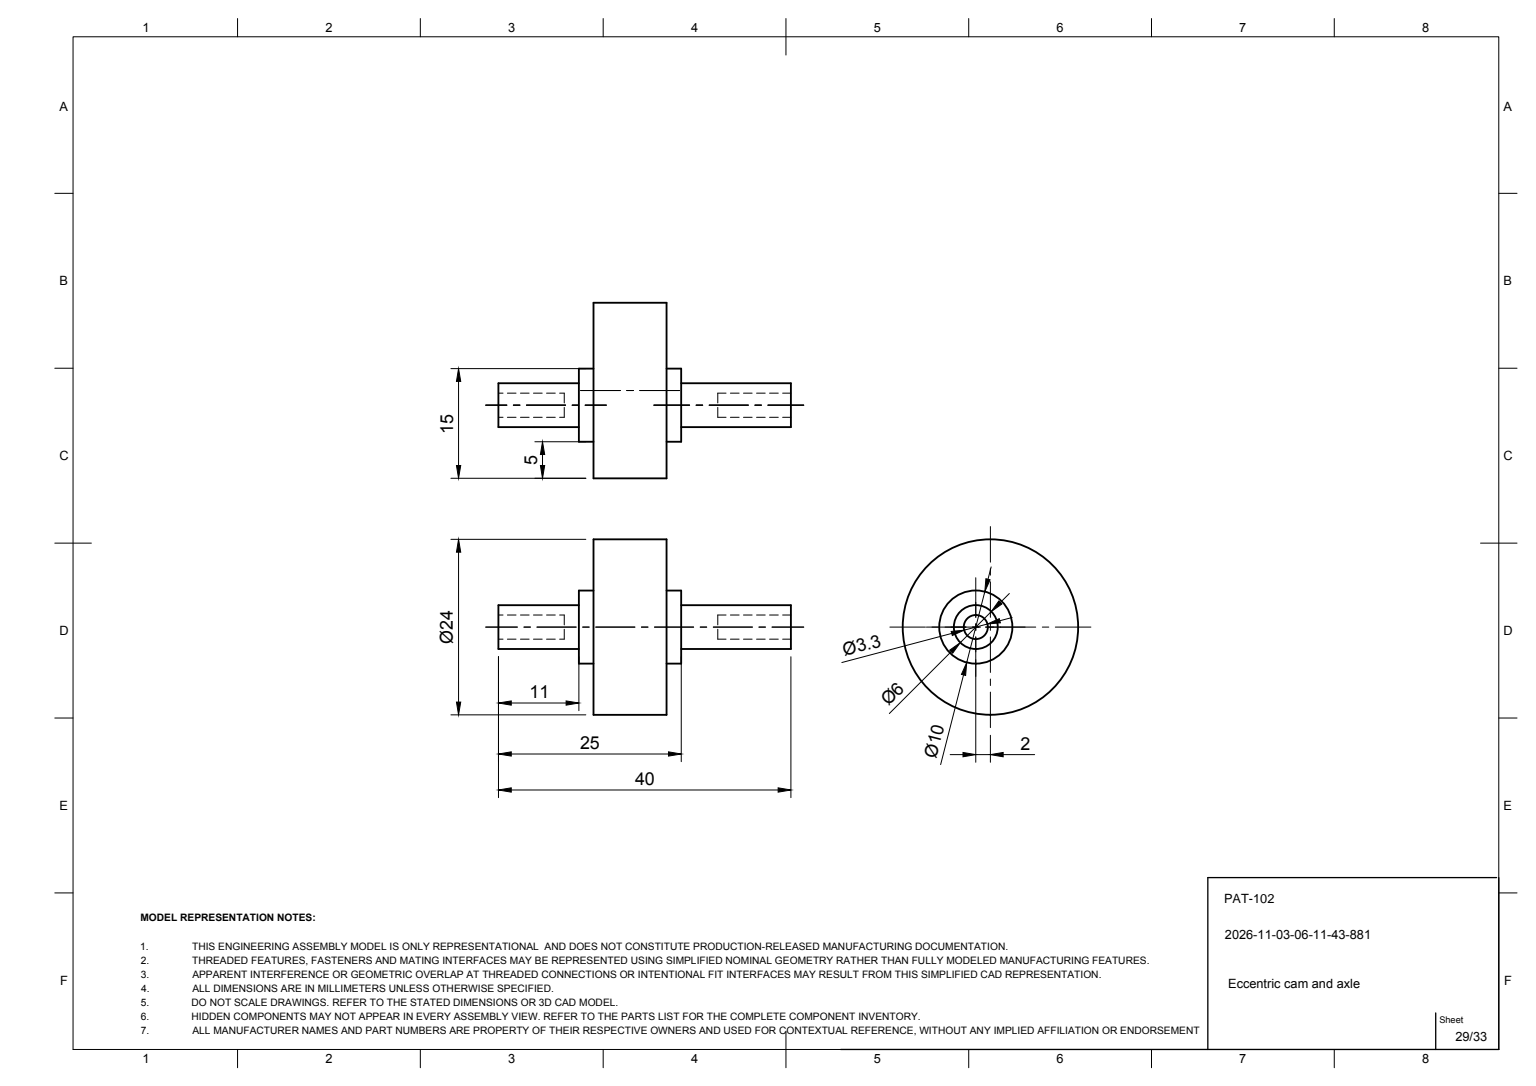
ISO-10303-21;
HEADER;
/* Generated by software containing ST-Developer
 * from STEP Tools, Inc. (www.steptools.com) 
 */

FILE_DESCRIPTION(
/* description */ ('Swing-away clamp arm'),
/* implementation_level */ '2;1');

FILE_NAME(
/* name */ 'Eccentric cam and axle.step',
/* time_stamp */ '2026-10-28T03:26:03-07:00',
/* author */ (''),
/* organization */ (''),
/* preprocessor_version */ 'ST-DEVELOPER v20.2',
/* originating_system */ 'Autodesk Translation Framework v15.17.0.0',
/* authorisation */ '');

FILE_SCHEMA (('AUTOMOTIVE_DESIGN { 1 0 10303 214 3 1 1 }'));
ENDSEC;

DATA;
#10=MECHANICAL_DESIGN_GEOMETRIC_PRESENTATION_REPRESENTATION('',(#320),#10627);
#260=SHAPE_REPRESENTATION_RELATIONSHIP('SRR','None',#10761,#286);
#286=ADVANCED_BREP_SHAPE_REPRESENTATION('',(#353),#10620);
#320=STYLED_ITEM('',(#10965),#353);
#353=MANIFOLD_SOLID_BREP('Body1',#4927);
#441=FACE_BOUND('',#1269,.T.);
#442=FACE_BOUND('',#1272,.T.);
#443=FACE_BOUND('',#1277,.T.);
#444=FACE_BOUND('',#1279,.T.);
#445=FACE_BOUND('',#1282,.T.);
#446=FACE_BOUND('',#1284,.T.);
#595=PLANE('',#5718);
#596=PLANE('',#5722);
#597=PLANE('',#5723);
#598=PLANE('',#5728);
#599=PLANE('',#5737);
#600=PLANE('',#5738);
#601=PLANE('',#5742);
#602=PLANE('',#5743);
#874=FACE_OUTER_BOUND('',#1264,.T.);
#875=FACE_OUTER_BOUND('',#1265,.T.);
#876=FACE_OUTER_BOUND('',#1266,.T.);
#877=FACE_OUTER_BOUND('',#1267,.T.);
#878=FACE_OUTER_BOUND('',#1268,.T.);
#879=FACE_OUTER_BOUND('',#1270,.T.);
#880=FACE_OUTER_BOUND('',#1271,.T.);
#881=FACE_OUTER_BOUND('',#1273,.T.);
#882=FACE_OUTER_BOUND('',#1274,.T.);
#883=FACE_OUTER_BOUND('',#1275,.T.);
#884=FACE_OUTER_BOUND('',#1276,.T.);
#885=FACE_OUTER_BOUND('',#1278,.T.);
#886=FACE_OUTER_BOUND('',#1280,.T.);
#887=FACE_OUTER_BOUND('',#1281,.T.);
#888=FACE_OUTER_BOUND('',#1283,.T.);
#1264=EDGE_LOOP('',(#4253,#4254,#4255,#4256));
#1265=EDGE_LOOP('',(#4257));
#1266=EDGE_LOOP('',(#4258,#4259,#4260,#4261));
#1267=EDGE_LOOP('',(#4262));
#1268=EDGE_LOOP('',(#4263));
#1269=EDGE_LOOP('',(#4264));
#1270=EDGE_LOOP('',(#4265,#4266,#4267,#4268));
#1271=EDGE_LOOP('',(#4269));
#1272=EDGE_LOOP('',(#4270));
#1273=EDGE_LOOP('',(#4271,#4272,#4273,#4274));
#1274=EDGE_LOOP('',(#4275,#4276,#4277,#4278));
#1275=EDGE_LOOP('',(#4279,#4280,#4281,#4282));
#1276=EDGE_LOOP('',(#4283));
#1277=EDGE_LOOP('',(#4284));
#1278=EDGE_LOOP('',(#4285));
#1279=EDGE_LOOP('',(#4286));
#1280=EDGE_LOOP('',(#4287,#4288,#4289,#4290));
#1281=EDGE_LOOP('',(#4291));
#1282=EDGE_LOOP('',(#4292));
#1283=EDGE_LOOP('',(#4293));
#1284=EDGE_LOOP('',(#4294));
#1602=LINE('',#10263,#1924);
#1603=LINE('',#10270,#1925);
#1604=LINE('',#10280,#1926);
#1605=LINE('',#10290,#1927);
#1606=LINE('',#10293,#1928);
#1607=LINE('',#10298,#1929);
#1608=LINE('',#10305,#1930);
#1924=VECTOR('',#7109,0.165);
#1925=VECTOR('',#7118,0.165);
#1926=VECTOR('',#7131,0.5);
#1927=VECTOR('',#7144,0.5);
#1928=VECTOR('',#7147,0.3);
#1929=VECTOR('',#7154,0.3);
#1930=VECTOR('',#7163,1.2);
#2211=CIRCLE('',#5716,0.165);
#2212=CIRCLE('',#5717,0.165);
#2213=CIRCLE('',#5720,0.165);
#2214=CIRCLE('',#5721,0.165);
#2215=CIRCLE('',#5724,0.5);
#2216=CIRCLE('',#5725,0.3);
#2217=CIRCLE('',#5727,0.5);
#2218=CIRCLE('',#5729,0.5);
#2219=CIRCLE('',#5730,0.3);
#2220=CIRCLE('',#5732,0.5);
#2221=CIRCLE('',#5734,0.3);
#2222=CIRCLE('',#5736,0.3);
#2223=CIRCLE('',#5740,1.2);
#2224=CIRCLE('',#5741,1.2);
#2594=VERTEX_POINT('',#10260);
#2595=VERTEX_POINT('',#10262);
#2596=VERTEX_POINT('',#10267);
#2597=VERTEX_POINT('',#10269);
#2598=VERTEX_POINT('',#10274);
#2599=VERTEX_POINT('',#10276);
#2600=VERTEX_POINT('',#10279);
#2601=VERTEX_POINT('',#10283);
#2602=VERTEX_POINT('',#10285);
#2603=VERTEX_POINT('',#10288);
#2604=VERTEX_POINT('',#10292);
#2605=VERTEX_POINT('',#10296);
#2606=VERTEX_POINT('',#10302);
#2607=VERTEX_POINT('',#10304);
#3159=EDGE_CURVE('',#2594,#2594,#2211,.T.);
#3160=EDGE_CURVE('',#2594,#2595,#1602,.T.);
#3161=EDGE_CURVE('',#2595,#2595,#2212,.T.);
#3162=EDGE_CURVE('',#2596,#2596,#2213,.T.);
#3163=EDGE_CURVE('',#2596,#2597,#1603,.T.);
#3164=EDGE_CURVE('',#2597,#2597,#2214,.T.);
#3165=EDGE_CURVE('',#2598,#2598,#2215,.T.);
#3166=EDGE_CURVE('',#2599,#2599,#2216,.T.);
#3167=EDGE_CURVE('',#2598,#2600,#1604,.T.);
#3168=EDGE_CURVE('',#2600,#2600,#2217,.T.);
#3169=EDGE_CURVE('',#2601,#2601,#2218,.T.);
#3170=EDGE_CURVE('',#2602,#2602,#2219,.T.);
#3171=EDGE_CURVE('',#2603,#2603,#2220,.T.);
#3172=EDGE_CURVE('',#2603,#2601,#1605,.T.);
#3173=EDGE_CURVE('',#2602,#2604,#1606,.T.);
#3174=EDGE_CURVE('',#2604,#2604,#2221,.T.);
#3175=EDGE_CURVE('',#2605,#2605,#2222,.T.);
#3176=EDGE_CURVE('',#2605,#2599,#1607,.T.);
#3177=EDGE_CURVE('',#2606,#2606,#2223,.T.);
#3178=EDGE_CURVE('',#2606,#2607,#1608,.T.);
#3179=EDGE_CURVE('',#2607,#2607,#2224,.T.);
#4253=ORIENTED_EDGE('',*,*,#3159,.F.);
#4254=ORIENTED_EDGE('',*,*,#3160,.T.);
#4255=ORIENTED_EDGE('',*,*,#3161,.F.);
#4256=ORIENTED_EDGE('',*,*,#3160,.F.);
#4257=ORIENTED_EDGE('',*,*,#3159,.T.);
#4258=ORIENTED_EDGE('',*,*,#3162,.F.);
#4259=ORIENTED_EDGE('',*,*,#3163,.T.);
#4260=ORIENTED_EDGE('',*,*,#3164,.T.);
#4261=ORIENTED_EDGE('',*,*,#3163,.F.);
#4262=ORIENTED_EDGE('',*,*,#3164,.F.);
#4263=ORIENTED_EDGE('',*,*,#3165,.T.);
#4264=ORIENTED_EDGE('',*,*,#3166,.F.);
#4265=ORIENTED_EDGE('',*,*,#3165,.F.);
#4266=ORIENTED_EDGE('',*,*,#3167,.T.);
#4267=ORIENTED_EDGE('',*,*,#3168,.F.);
#4268=ORIENTED_EDGE('',*,*,#3167,.F.);
#4269=ORIENTED_EDGE('',*,*,#3169,.F.);
#4270=ORIENTED_EDGE('',*,*,#3170,.F.);
#4271=ORIENTED_EDGE('',*,*,#3171,.F.);
#4272=ORIENTED_EDGE('',*,*,#3172,.T.);
#4273=ORIENTED_EDGE('',*,*,#3169,.T.);
#4274=ORIENTED_EDGE('',*,*,#3172,.F.);
#4275=ORIENTED_EDGE('',*,*,#3170,.T.);
#4276=ORIENTED_EDGE('',*,*,#3173,.T.);
#4277=ORIENTED_EDGE('',*,*,#3174,.T.);
#4278=ORIENTED_EDGE('',*,*,#3173,.F.);
#4279=ORIENTED_EDGE('',*,*,#3175,.F.);
#4280=ORIENTED_EDGE('',*,*,#3176,.T.);
#4281=ORIENTED_EDGE('',*,*,#3166,.T.);
#4282=ORIENTED_EDGE('',*,*,#3176,.F.);
#4283=ORIENTED_EDGE('',*,*,#3175,.T.);
#4284=ORIENTED_EDGE('',*,*,#3161,.T.);
#4285=ORIENTED_EDGE('',*,*,#3174,.F.);
#4286=ORIENTED_EDGE('',*,*,#3162,.T.);
#4287=ORIENTED_EDGE('',*,*,#3177,.F.);
#4288=ORIENTED_EDGE('',*,*,#3178,.T.);
#4289=ORIENTED_EDGE('',*,*,#3179,.T.);
#4290=ORIENTED_EDGE('',*,*,#3178,.F.);
#4291=ORIENTED_EDGE('',*,*,#3177,.T.);
#4292=ORIENTED_EDGE('',*,*,#3168,.T.);
#4293=ORIENTED_EDGE('',*,*,#3179,.F.);
#4294=ORIENTED_EDGE('',*,*,#3171,.T.);
#4571=CYLINDRICAL_SURFACE('',#5715,0.165);
#4572=CYLINDRICAL_SURFACE('',#5719,0.165);
#4573=CYLINDRICAL_SURFACE('',#5726,0.5);
#4574=CYLINDRICAL_SURFACE('',#5731,0.5);
#4575=CYLINDRICAL_SURFACE('',#5733,0.3);
#4576=CYLINDRICAL_SURFACE('',#5735,0.3);
#4577=CYLINDRICAL_SURFACE('',#5739,1.2);
#4829=ADVANCED_FACE('',(#874),#4571,.F.);
#4830=ADVANCED_FACE('',(#875),#595,.T.);
#4831=ADVANCED_FACE('',(#876),#4572,.F.);
#4832=ADVANCED_FACE('',(#877),#596,.F.);
#4833=ADVANCED_FACE('',(#878,#441),#597,.T.);
#4834=ADVANCED_FACE('',(#879),#4573,.T.);
#4835=ADVANCED_FACE('',(#880,#442),#598,.F.);
#4836=ADVANCED_FACE('',(#881),#4574,.T.);
#4837=ADVANCED_FACE('',(#882),#4575,.T.);
#4838=ADVANCED_FACE('',(#883),#4576,.T.);
#4839=ADVANCED_FACE('',(#884,#443),#599,.T.);
#4840=ADVANCED_FACE('',(#885,#444),#600,.F.);
#4841=ADVANCED_FACE('',(#886),#4577,.T.);
#4842=ADVANCED_FACE('',(#887,#445),#601,.T.);
#4843=ADVANCED_FACE('',(#888,#446),#602,.F.);
#4927=CLOSED_SHELL('',(#4829,#4830,#4831,#4832,#4833,#4834,#4835,#4836,
#4837,#4838,#4839,#4840,#4841,#4842,#4843));
#5714=AXIS2_PLACEMENT_3D('',#10258,#7103,#7104);
#5715=AXIS2_PLACEMENT_3D('',#10259,#7105,#7106);
#5716=AXIS2_PLACEMENT_3D('',#10261,#7107,#7108);
#5717=AXIS2_PLACEMENT_3D('',#10264,#7110,#7111);
#5718=AXIS2_PLACEMENT_3D('',#10265,#7112,#7113);
#5719=AXIS2_PLACEMENT_3D('',#10266,#7114,#7115);
#5720=AXIS2_PLACEMENT_3D('',#10268,#7116,#7117);
#5721=AXIS2_PLACEMENT_3D('',#10271,#7119,#7120);
#5722=AXIS2_PLACEMENT_3D('',#10272,#7121,#7122);
#5723=AXIS2_PLACEMENT_3D('',#10273,#7123,#7124);
#5724=AXIS2_PLACEMENT_3D('',#10275,#7125,#7126);
#5725=AXIS2_PLACEMENT_3D('',#10277,#7127,#7128);
#5726=AXIS2_PLACEMENT_3D('',#10278,#7129,#7130);
#5727=AXIS2_PLACEMENT_3D('',#10281,#7132,#7133);
#5728=AXIS2_PLACEMENT_3D('',#10282,#7134,#7135);
#5729=AXIS2_PLACEMENT_3D('',#10284,#7136,#7137);
#5730=AXIS2_PLACEMENT_3D('',#10286,#7138,#7139);
#5731=AXIS2_PLACEMENT_3D('',#10287,#7140,#7141);
#5732=AXIS2_PLACEMENT_3D('',#10289,#7142,#7143);
#5733=AXIS2_PLACEMENT_3D('',#10291,#7145,#7146);
#5734=AXIS2_PLACEMENT_3D('',#10294,#7148,#7149);
#5735=AXIS2_PLACEMENT_3D('',#10295,#7150,#7151);
#5736=AXIS2_PLACEMENT_3D('',#10297,#7152,#7153);
#5737=AXIS2_PLACEMENT_3D('',#10299,#7155,#7156);
#5738=AXIS2_PLACEMENT_3D('',#10300,#7157,#7158);
#5739=AXIS2_PLACEMENT_3D('',#10301,#7159,#7160);
#5740=AXIS2_PLACEMENT_3D('',#10303,#7161,#7162);
#5741=AXIS2_PLACEMENT_3D('',#10306,#7164,#7165);
#5742=AXIS2_PLACEMENT_3D('',#10307,#7166,#7167);
#5743=AXIS2_PLACEMENT_3D('',#10308,#7168,#7169);
#7103=DIRECTION('axis',(0.,0.,1.));
#7104=DIRECTION('refdir',(1.,0.,0.));
#7105=DIRECTION('center_axis',(0.,1.,0.));
#7106=DIRECTION('ref_axis',(1.,0.,0.));
#7107=DIRECTION('center_axis',(0.,1.,0.));
#7108=DIRECTION('ref_axis',(1.,0.,0.));
#7109=DIRECTION('',(0.,1.,0.));
#7110=DIRECTION('center_axis',(0.,-1.,0.));
#7111=DIRECTION('ref_axis',(1.,0.,0.));
#7112=DIRECTION('center_axis',(0.,1.,0.));
#7113=DIRECTION('ref_axis',(1.,0.,0.));
#7114=DIRECTION('center_axis',(0.,1.,0.));
#7115=DIRECTION('ref_axis',(1.,0.,0.));
#7116=DIRECTION('center_axis',(0.,1.,0.));
#7117=DIRECTION('ref_axis',(1.,0.,0.));
#7118=DIRECTION('',(0.,1.,0.));
#7119=DIRECTION('center_axis',(0.,1.,0.));
#7120=DIRECTION('ref_axis',(1.,0.,0.));
#7121=DIRECTION('center_axis',(0.,1.,0.));
#7122=DIRECTION('ref_axis',(1.,0.,0.));
#7123=DIRECTION('center_axis',(0.,1.,0.));
#7124=DIRECTION('ref_axis',(1.,0.,0.));
#7125=DIRECTION('center_axis',(0.,1.,0.));
#7126=DIRECTION('ref_axis',(1.,0.,0.));
#7127=DIRECTION('center_axis',(0.,1.,0.));
#7128=DIRECTION('ref_axis',(1.,0.,0.));
#7129=DIRECTION('center_axis',(0.,1.,0.));
#7130=DIRECTION('ref_axis',(1.,0.,0.));
#7131=DIRECTION('',(0.,-1.,0.));
#7132=DIRECTION('center_axis',(0.,-1.,0.));
#7133=DIRECTION('ref_axis',(1.,0.,0.));
#7134=DIRECTION('center_axis',(0.,1.,0.));
#7135=DIRECTION('ref_axis',(1.,0.,0.));
#7136=DIRECTION('center_axis',(0.,1.,0.));
#7137=DIRECTION('ref_axis',(1.,0.,0.));
#7138=DIRECTION('center_axis',(0.,-1.,0.));
#7139=DIRECTION('ref_axis',(1.,0.,0.));
#7140=DIRECTION('center_axis',(0.,1.,0.));
#7141=DIRECTION('ref_axis',(1.,0.,0.));
#7142=DIRECTION('center_axis',(0.,1.,0.));
#7143=DIRECTION('ref_axis',(1.,0.,0.));
#7144=DIRECTION('',(0.,-1.,0.));
#7145=DIRECTION('center_axis',(0.,1.,0.));
#7146=DIRECTION('ref_axis',(1.,0.,0.));
#7147=DIRECTION('',(0.,-1.,0.));
#7148=DIRECTION('center_axis',(0.,1.,0.));
#7149=DIRECTION('ref_axis',(1.,0.,0.));
#7150=DIRECTION('center_axis',(0.,1.,0.));
#7151=DIRECTION('ref_axis',(1.,0.,0.));
#7152=DIRECTION('center_axis',(0.,1.,0.));
#7153=DIRECTION('ref_axis',(1.,0.,0.));
#7154=DIRECTION('',(0.,-1.,0.));
#7155=DIRECTION('center_axis',(0.,1.,0.));
#7156=DIRECTION('ref_axis',(1.,0.,0.));
#7157=DIRECTION('center_axis',(0.,1.,0.));
#7158=DIRECTION('ref_axis',(1.,0.,0.));
#7159=DIRECTION('center_axis',(0.,1.,0.));
#7160=DIRECTION('ref_axis',(1.,0.,0.));
#7161=DIRECTION('center_axis',(0.,1.,0.));
#7162=DIRECTION('ref_axis',(1.,0.,0.));
#7163=DIRECTION('',(0.,-1.,0.));
#7164=DIRECTION('center_axis',(0.,1.,0.));
#7165=DIRECTION('ref_axis',(1.,0.,0.));
#7166=DIRECTION('center_axis',(0.,1.,0.));
#7167=DIRECTION('ref_axis',(1.,0.,0.));
#7168=DIRECTION('center_axis',(0.,1.,0.));
#7169=DIRECTION('ref_axis',(1.,0.,0.));
#10258=CARTESIAN_POINT('',(0.,0.,0.));
#10259=CARTESIAN_POINT('Origin',(2.,0.9,10.5));
#10260=CARTESIAN_POINT('',(1.835,0.9,10.5));
#10261=CARTESIAN_POINT('Origin',(2.,0.9,10.5));
#10262=CARTESIAN_POINT('',(1.835,1.8,10.5));
#10263=CARTESIAN_POINT('',(1.835,0.9,10.5));
#10264=CARTESIAN_POINT('Origin',(2.,1.8,10.5));
#10265=CARTESIAN_POINT('Origin',(2.,0.9,10.5));
#10266=CARTESIAN_POINT('Origin',(2.,-2.3,10.5));
#10267=CARTESIAN_POINT('',(1.835,-2.2,10.5));
#10268=CARTESIAN_POINT('Origin',(2.,-2.2,10.5));
#10269=CARTESIAN_POINT('',(1.835,-1.2,10.5));
#10270=CARTESIAN_POINT('',(1.835,-2.3,10.5));
#10271=CARTESIAN_POINT('Origin',(2.,-1.2,10.5));
#10272=CARTESIAN_POINT('Origin',(2.,-1.2,10.5));
#10273=CARTESIAN_POINT('Origin',(2.,0.7,10.5));
#10274=CARTESIAN_POINT('',(1.5,0.7,10.5));
#10275=CARTESIAN_POINT('Origin',(2.,0.7,10.5));
#10276=CARTESIAN_POINT('',(1.7,0.7,10.5));
#10277=CARTESIAN_POINT('Origin',(2.,0.7,10.5));
#10278=CARTESIAN_POINT('Origin',(2.,0.5,10.5));
#10279=CARTESIAN_POINT('',(1.5,0.5,10.5));
#10280=CARTESIAN_POINT('',(1.5,0.5,10.5));
#10281=CARTESIAN_POINT('Origin',(2.,0.5,10.5));
#10282=CARTESIAN_POINT('Origin',(2.,-0.7,10.5));
#10283=CARTESIAN_POINT('',(1.5,-0.7,10.5));
#10284=CARTESIAN_POINT('Origin',(2.,-0.7,10.5));
#10285=CARTESIAN_POINT('',(1.7,-0.7,10.5));
#10286=CARTESIAN_POINT('Origin',(2.,-0.7,10.5));
#10287=CARTESIAN_POINT('Origin',(2.,-0.7,10.5));
#10288=CARTESIAN_POINT('',(1.5,-0.5,10.5));
#10289=CARTESIAN_POINT('Origin',(2.,-0.5,10.5));
#10290=CARTESIAN_POINT('',(1.5,-0.7,10.5));
#10291=CARTESIAN_POINT('Origin',(2.,-2.2,10.5));
#10292=CARTESIAN_POINT('',(1.7,-2.2,10.5));
#10293=CARTESIAN_POINT('',(1.7,-2.2,10.5));
#10294=CARTESIAN_POINT('Origin',(2.,-2.2,10.5));
#10295=CARTESIAN_POINT('Origin',(2.,-2.2,10.5));
#10296=CARTESIAN_POINT('',(1.7,1.8,10.5));
#10297=CARTESIAN_POINT('Origin',(2.,1.8,10.5));
#10298=CARTESIAN_POINT('',(1.7,-2.2,10.5));
#10299=CARTESIAN_POINT('Origin',(2.,1.8,10.5));
#10300=CARTESIAN_POINT('Origin',(2.,-2.2,10.5));
#10301=CARTESIAN_POINT('Origin',(2.,-0.5,10.7));
#10302=CARTESIAN_POINT('',(0.8,0.5,10.7));
#10303=CARTESIAN_POINT('Origin',(2.,0.5,10.7));
#10304=CARTESIAN_POINT('',(0.8,-0.5,10.7));
#10305=CARTESIAN_POINT('',(0.8,-0.5,10.7));
#10306=CARTESIAN_POINT('Origin',(2.,-0.5,10.7));
#10307=CARTESIAN_POINT('Origin',(2.,0.5,10.7));
#10308=CARTESIAN_POINT('Origin',(2.,-0.5,10.7));
#10588=UNCERTAINTY_MEASURE_WITH_UNIT(LENGTH_MEASURE(0.001),#10628,
'DISTANCE_ACCURACY_VALUE',
'Maximum model space distance between geometric entities at asserted c
onnectivities');
#10595=UNCERTAINTY_MEASURE_WITH_UNIT(LENGTH_MEASURE(0.001),#10628,
'DISTANCE_ACCURACY_VALUE',
'Maximum model space distance between geometric entities at asserted c
onnectivities');
#10620=(
GEOMETRIC_REPRESENTATION_CONTEXT(3)
GLOBAL_UNCERTAINTY_ASSIGNED_CONTEXT((#10588))
GLOBAL_UNIT_ASSIGNED_CONTEXT((#10628,#10630,#10631))
REPRESENTATION_CONTEXT('','3D')
);
#10627=(
GEOMETRIC_REPRESENTATION_CONTEXT(3)
GLOBAL_UNCERTAINTY_ASSIGNED_CONTEXT((#10595))
GLOBAL_UNIT_ASSIGNED_CONTEXT((#10628,#10630,#10631))
REPRESENTATION_CONTEXT('','3D')
);
#10628=(
LENGTH_UNIT()
NAMED_UNIT(*)
SI_UNIT(.CENTI.,.METRE.)
);
#10630=(
NAMED_UNIT(*)
PLANE_ANGLE_UNIT()
SI_UNIT($,.RADIAN.)
);
#10631=(
NAMED_UNIT(*)
SI_UNIT($,.STERADIAN.)
SOLID_ANGLE_UNIT()
);
#10656=SHAPE_DEFINITION_REPRESENTATION(#10702,#10761);
#10702=PRODUCT_DEFINITION_SHAPE('',$,#10793);
#10761=SHAPE_REPRESENTATION('',(#5714),#10620);
#10768=PRODUCT_DEFINITION_CONTEXT('part definition',#10863,'design');
#10793=PRODUCT_DEFINITION('Eccentric cam and axle',
'Eccentric cam and axle',#10824,#10768);
#10824=PRODUCT_DEFINITION_FORMATION('',$,#10889);
#10863=APPLICATION_CONTEXT(
'Core Data for Automotive Mechanical Design Process');
#10864=PRODUCT_CONTEXT('part definition',#10863,'mechanical');
#10889=PRODUCT('Eccentric cam and axle','Eccentric cam and axle',
'Eccentric cam and axle',(#10864));
#10959=COLOUR_RGB('Grey',0.48,0.52,0.57);
#10960=FILL_AREA_STYLE_COLOUR('',#10959);
#10961=FILL_AREA_STYLE('',(#10960));
#10962=SURFACE_STYLE_FILL_AREA(#10961);
#10963=SURFACE_SIDE_STYLE('',(#10962));
#10964=SURFACE_STYLE_USAGE(.BOTH.,#10963);
#10965=PRESENTATION_STYLE_ASSIGNMENT((#10964));
ENDSEC;
END-ISO-10303-21;
